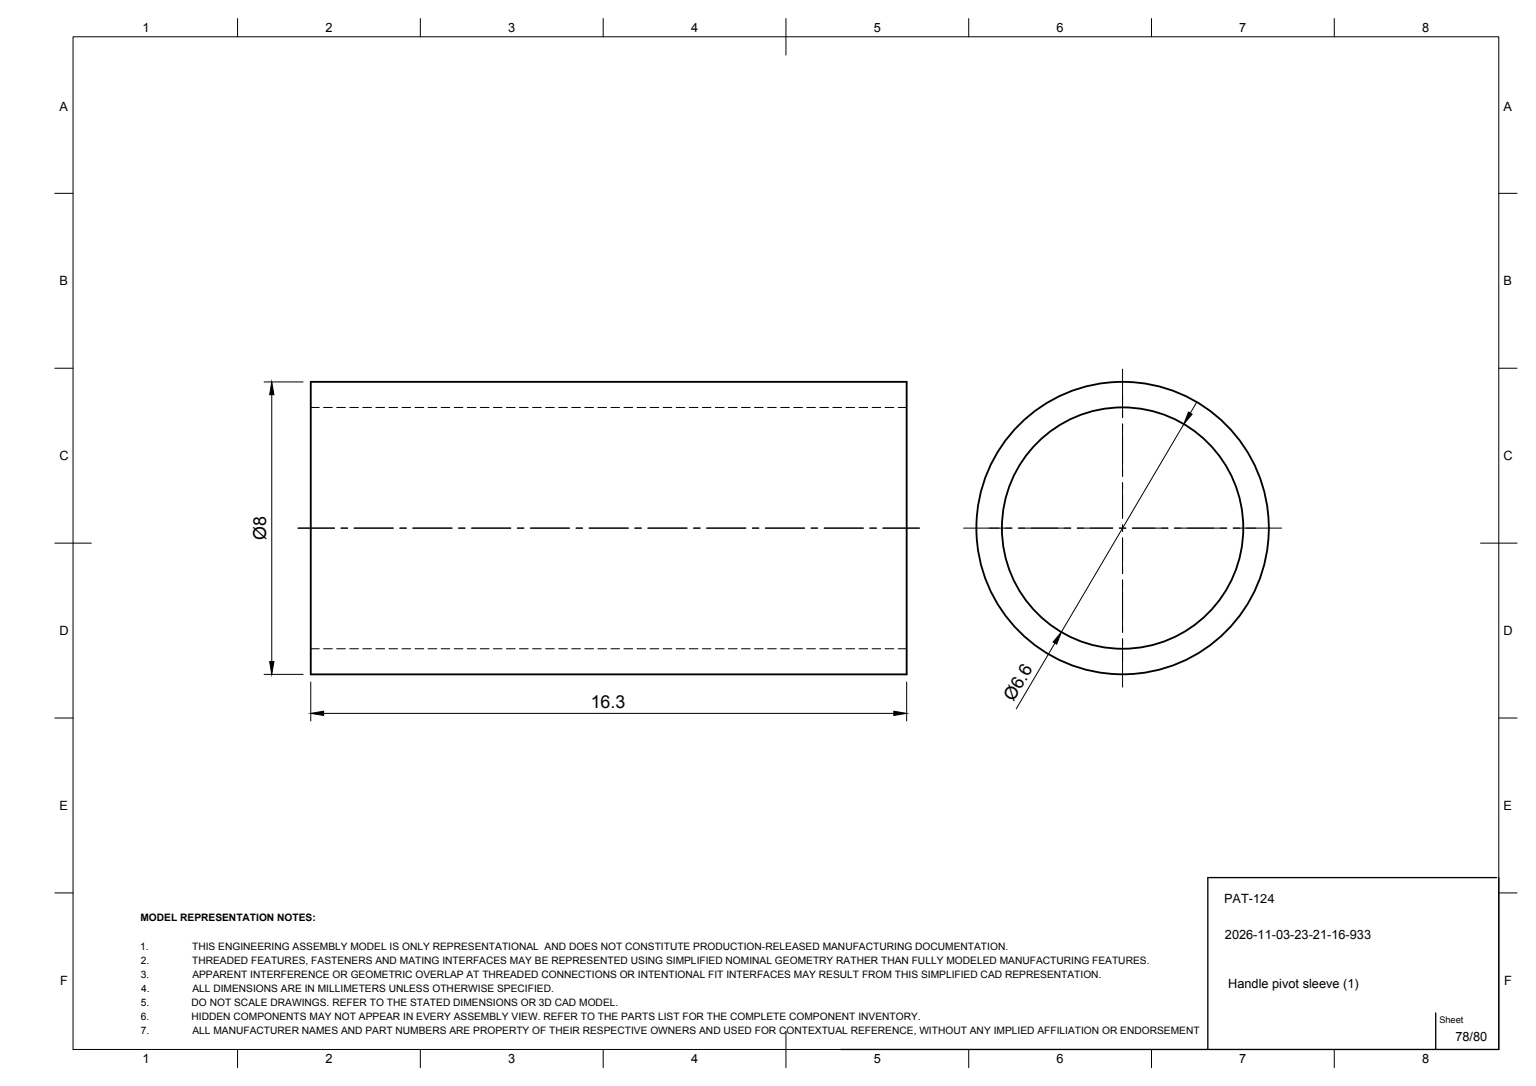
ISO-10303-21;
HEADER;
/* Generated by software containing ST-Developer
 * from STEP Tools, Inc. (www.steptools.com) 
 */

FILE_DESCRIPTION(
/* description */ ('XY cross-slide table'),
/* implementation_level */ '2;1');

FILE_NAME(
/* name */ 'Handle pivot sleeve (1).step',
/* time_stamp */ '2026-10-28T03:22:46-07:00',
/* author */ (''),
/* organization */ (''),
/* preprocessor_version */ 'ST-DEVELOPER v20.2',
/* originating_system */ 'Autodesk Translation Framework v15.17.0.0',
/* authorisation */ '');

FILE_SCHEMA (('AUTOMOTIVE_DESIGN { 1 0 10303 214 3 1 1 }'));
ENDSEC;

DATA;
#10=MECHANICAL_DESIGN_GEOMETRIC_PRESENTATION_REPRESENTATION('',(#1777),#62984);
#1581=SHAPE_REPRESENTATION_RELATIONSHIP('SRR','None',#63441,#1664);
#1664=ADVANCED_BREP_SHAPE_REPRESENTATION('',(#1882),#62978);
#1777=STYLED_ITEM('',(#63905),#1882);
#1882=MANIFOLD_SOLID_BREP('Body1',#23079);
#2288=FACE_BOUND('',#5850,.T.);
#2289=FACE_BOUND('',#5852,.T.);
#2833=PLANE('',#26336);
#2834=PLANE('',#26337);
#4132=FACE_OUTER_BOUND('',#5847,.T.);
#4133=FACE_OUTER_BOUND('',#5848,.T.);
#4134=FACE_OUTER_BOUND('',#5849,.T.);
#4135=FACE_OUTER_BOUND('',#5851,.T.);
#5847=EDGE_LOOP('',(#20842,#20843,#20844,#20845));
#5848=EDGE_LOOP('',(#20846,#20847,#20848,#20849));
#5849=EDGE_LOOP('',(#20850));
#5850=EDGE_LOOP('',(#20851));
#5851=EDGE_LOOP('',(#20852));
#5852=EDGE_LOOP('',(#20853));
#7318=LINE('',#62521,#8805);
#7319=LINE('',#62527,#8806);
#8805=VECTOR('',#32537,0.33);
#8806=VECTOR('',#32544,0.4);
#9749=CIRCLE('',#26331,0.33);
#9750=CIRCLE('',#26332,0.33);
#9751=CIRCLE('',#26334,0.4);
#9752=CIRCLE('',#26335,0.4);
#11772=VERTEX_POINT('',#62518);
#11773=VERTEX_POINT('',#62520);
#11774=VERTEX_POINT('',#62524);
#11775=VERTEX_POINT('',#62526);
#14805=EDGE_CURVE('',#11772,#11772,#9749,.T.);
#14806=EDGE_CURVE('',#11772,#11773,#7318,.T.);
#14807=EDGE_CURVE('',#11773,#11773,#9750,.T.);
#14808=EDGE_CURVE('',#11774,#11774,#9751,.T.);
#14809=EDGE_CURVE('',#11774,#11775,#7319,.T.);
#14810=EDGE_CURVE('',#11775,#11775,#9752,.T.);
#20842=ORIENTED_EDGE('',*,*,#14805,.F.);
#20843=ORIENTED_EDGE('',*,*,#14806,.T.);
#20844=ORIENTED_EDGE('',*,*,#14807,.T.);
#20845=ORIENTED_EDGE('',*,*,#14806,.F.);
#20846=ORIENTED_EDGE('',*,*,#14808,.F.);
#20847=ORIENTED_EDGE('',*,*,#14809,.T.);
#20848=ORIENTED_EDGE('',*,*,#14810,.T.);
#20849=ORIENTED_EDGE('',*,*,#14809,.F.);
#20850=ORIENTED_EDGE('',*,*,#14808,.T.);
#20851=ORIENTED_EDGE('',*,*,#14805,.T.);
#20852=ORIENTED_EDGE('',*,*,#14810,.F.);
#20853=ORIENTED_EDGE('',*,*,#14807,.F.);
#21641=CYLINDRICAL_SURFACE('',#26330,0.33);
#21642=CYLINDRICAL_SURFACE('',#26333,0.4);
#22913=ADVANCED_FACE('',(#4132),#21641,.F.);
#22914=ADVANCED_FACE('',(#4133),#21642,.T.);
#22915=ADVANCED_FACE('',(#4134,#2288),#2833,.T.);
#22916=ADVANCED_FACE('',(#4135,#2289),#2834,.F.);
#23079=CLOSED_SHELL('',(#22913,#22914,#22915,#22916));
#26329=AXIS2_PLACEMENT_3D('',#62516,#32531,#32532);
#26330=AXIS2_PLACEMENT_3D('',#62517,#32533,#32534);
#26331=AXIS2_PLACEMENT_3D('',#62519,#32535,#32536);
#26332=AXIS2_PLACEMENT_3D('',#62522,#32538,#32539);
#26333=AXIS2_PLACEMENT_3D('',#62523,#32540,#32541);
#26334=AXIS2_PLACEMENT_3D('',#62525,#32542,#32543);
#26335=AXIS2_PLACEMENT_3D('',#62528,#32545,#32546);
#26336=AXIS2_PLACEMENT_3D('',#62529,#32547,#32548);
#26337=AXIS2_PLACEMENT_3D('',#62530,#32549,#32550);
#32531=DIRECTION('axis',(0.,0.,1.));
#32532=DIRECTION('refdir',(1.,0.,0.));
#32533=DIRECTION('center_axis',(1.,0.,0.));
#32534=DIRECTION('ref_axis',(0.,0.,-1.));
#32535=DIRECTION('center_axis',(-1.,0.,0.));
#32536=DIRECTION('ref_axis',(0.,0.,-1.));
#32537=DIRECTION('',(-1.,0.,0.));
#32538=DIRECTION('center_axis',(-1.,0.,0.));
#32539=DIRECTION('ref_axis',(0.,0.,-1.));
#32540=DIRECTION('center_axis',(1.,0.,0.));
#32541=DIRECTION('ref_axis',(0.,0.,-1.));
#32542=DIRECTION('center_axis',(1.,0.,0.));
#32543=DIRECTION('ref_axis',(0.,0.,-1.));
#32544=DIRECTION('',(-1.,0.,0.));
#32545=DIRECTION('center_axis',(1.,0.,0.));
#32546=DIRECTION('ref_axis',(0.,0.,-1.));
#32547=DIRECTION('center_axis',(1.,0.,0.));
#32548=DIRECTION('ref_axis',(0.,0.,-1.));
#32549=DIRECTION('center_axis',(1.,0.,0.));
#32550=DIRECTION('ref_axis',(0.,0.,-1.));
#62516=CARTESIAN_POINT('',(0.,0.,0.));
#62517=CARTESIAN_POINT('Origin',(29.4,0.,6.5));
#62518=CARTESIAN_POINT('',(31.03,-4.04133443718627E-17,6.83));
#62519=CARTESIAN_POINT('Origin',(31.03,0.,6.5));
#62520=CARTESIAN_POINT('',(29.4,-4.04133443718627E-17,6.83));
#62521=CARTESIAN_POINT('',(29.4,-4.04133443718627E-17,6.83));
#62522=CARTESIAN_POINT('Origin',(29.4,0.,6.5));
#62523=CARTESIAN_POINT('Origin',(29.4,0.,6.5));
#62524=CARTESIAN_POINT('',(31.03,-4.89858719658942E-17,6.9));
#62525=CARTESIAN_POINT('Origin',(31.03,0.,6.5));
#62526=CARTESIAN_POINT('',(29.4,-4.89858719658942E-17,6.9));
#62527=CARTESIAN_POINT('',(29.4,-4.89858719658942E-17,6.9));
#62528=CARTESIAN_POINT('Origin',(29.4,0.,6.5));
#62529=CARTESIAN_POINT('Origin',(31.03,0.,6.5));
#62530=CARTESIAN_POINT('Origin',(29.4,0.,6.5));
#62879=UNCERTAINTY_MEASURE_WITH_UNIT(LENGTH_MEASURE(0.001),#62985,
'DISTANCE_ACCURACY_VALUE',
'Maximum model space distance between geometric entities at asserted c
onnectivities');
#62885=UNCERTAINTY_MEASURE_WITH_UNIT(LENGTH_MEASURE(0.001),#62985,
'DISTANCE_ACCURACY_VALUE',
'Maximum model space distance between geometric entities at asserted c
onnectivities');
#62978=(
GEOMETRIC_REPRESENTATION_CONTEXT(3)
GLOBAL_UNCERTAINTY_ASSIGNED_CONTEXT((#62879))
GLOBAL_UNIT_ASSIGNED_CONTEXT((#62985,#62987,#62988))
REPRESENTATION_CONTEXT('','3D')
);
#62984=(
GEOMETRIC_REPRESENTATION_CONTEXT(3)
GLOBAL_UNCERTAINTY_ASSIGNED_CONTEXT((#62885))
GLOBAL_UNIT_ASSIGNED_CONTEXT((#62985,#62987,#62988))
REPRESENTATION_CONTEXT('','3D')
);
#62985=(
LENGTH_UNIT()
NAMED_UNIT(*)
SI_UNIT(.CENTI.,.METRE.)
);
#62987=(
NAMED_UNIT(*)
PLANE_ANGLE_UNIT()
SI_UNIT($,.RADIAN.)
);
#62988=(
NAMED_UNIT(*)
SI_UNIT($,.STERADIAN.)
SOLID_ANGLE_UNIT()
);
#63081=SHAPE_DEFINITION_REPRESENTATION(#63292,#63441);
#63292=PRODUCT_DEFINITION_SHAPE('',$,#63540);
#63441=SHAPE_REPRESENTATION('',(#26329),#62978);
#63447=PRODUCT_DEFINITION_CONTEXT('part definition',#63743,'design');
#63540=PRODUCT_DEFINITION('Handle pivot sleeve (1)',
'Handle pivot sleeve (1)',#63638,#63447);
#63638=PRODUCT_DEFINITION_FORMATION('',$,#63837);
#63743=APPLICATION_CONTEXT(
'Core Data for Automotive Mechanical Design Process');
#63744=PRODUCT_CONTEXT('part definition',#63743,'mechanical');
#63837=PRODUCT('Handle pivot sleeve (1)','Handle pivot sleeve (1)',
'Handle pivot sleeve (1)',(#63744));
#63899=COLOUR_RGB('Sky Blue',0.24,0.69,0.87);
#63900=FILL_AREA_STYLE_COLOUR('',#63899);
#63901=FILL_AREA_STYLE('',(#63900));
#63902=SURFACE_STYLE_FILL_AREA(#63901);
#63903=SURFACE_SIDE_STYLE('',(#63902));
#63904=SURFACE_STYLE_USAGE(.BOTH.,#63903);
#63905=PRESENTATION_STYLE_ASSIGNMENT((#63904));
ENDSEC;
END-ISO-10303-21;
